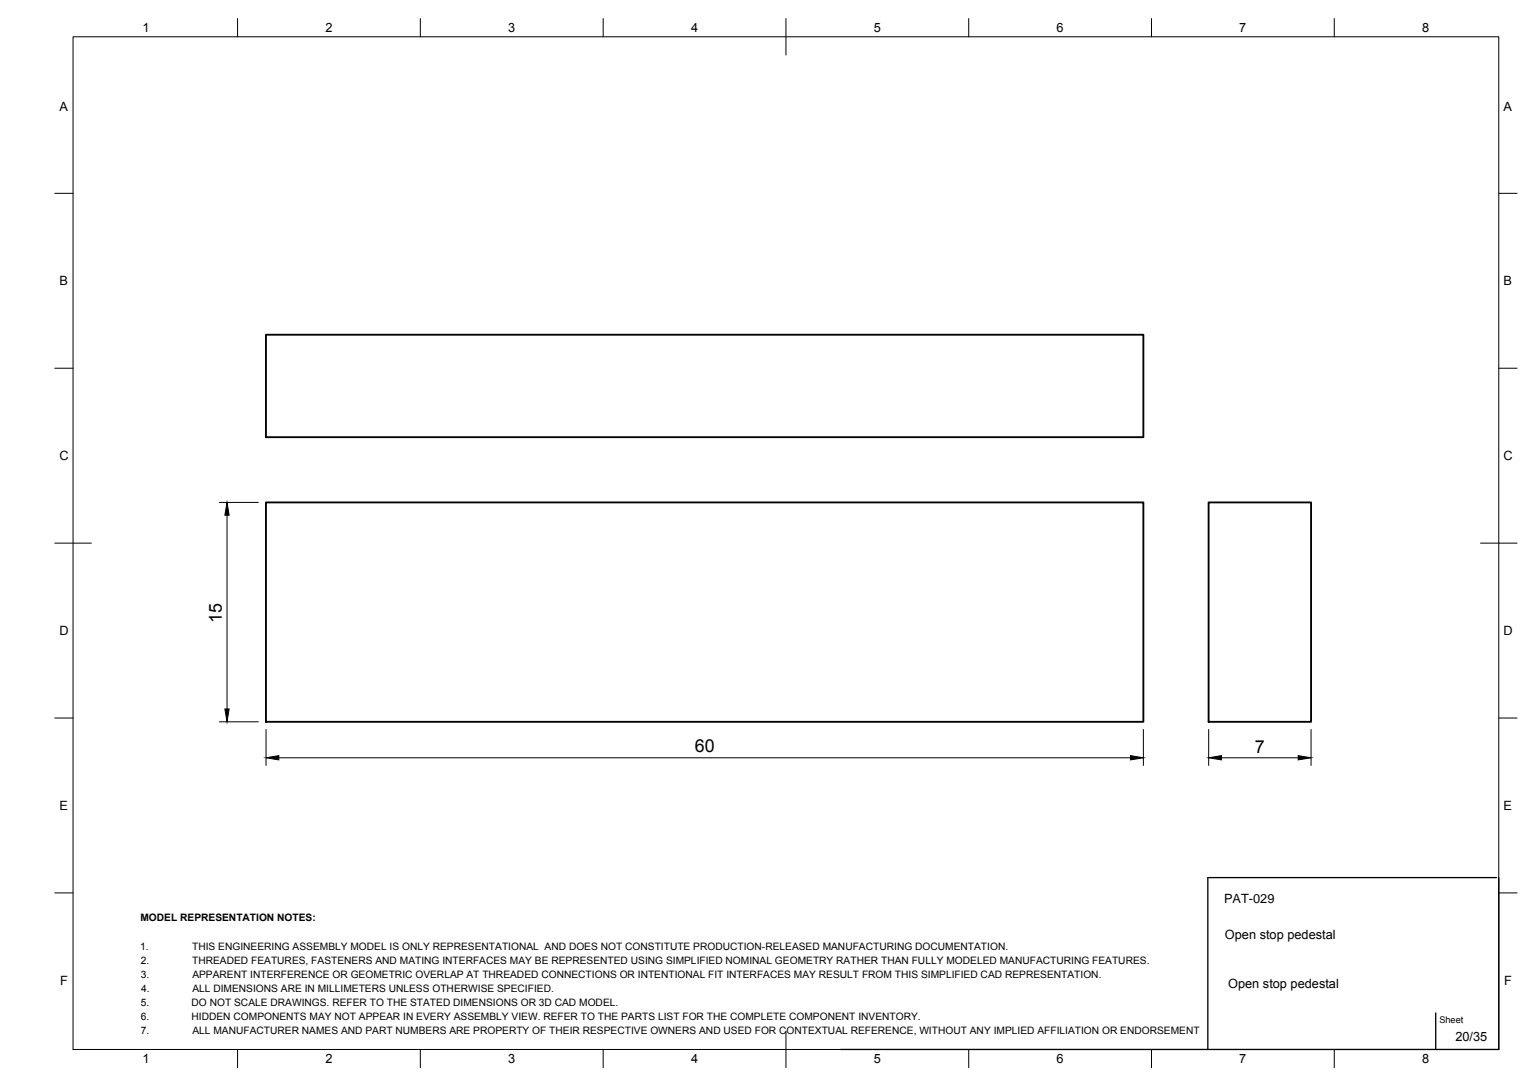
ISO-10303-21;
HEADER;
/* Generated by software containing ST-Developer
 * from STEP Tools, Inc. (www.steptools.com) 
 */

FILE_DESCRIPTION(
/* description */ ('Door-style hinge test fixture with detent'),
/* implementation_level */ '2;1');

FILE_NAME(
/* name */ 'Open stop pedestal.step',
/* time_stamp */ '2026-10-28T03:24:57-07:00',
/* author */ (''),
/* organization */ (''),
/* preprocessor_version */ 'ST-DEVELOPER v20.2',
/* originating_system */ 'Autodesk Translation Framework v15.17.0.0',
/* authorisation */ '');

FILE_SCHEMA (('AUTOMOTIVE_DESIGN { 1 0 10303 214 3 1 1 }'));
ENDSEC;

DATA;
#10=MECHANICAL_DESIGN_GEOMETRIC_PRESENTATION_REPRESENTATION('',(#338),#9813);
#275=SHAPE_REPRESENTATION_RELATIONSHIP('SRR','None',#9952,#306);
#306=ADVANCED_BREP_SHAPE_REPRESENTATION('',(#378),#9795);
#338=STYLED_ITEM('',(#10169),#378);
#378=MANIFOLD_SOLID_BREP('Body1',#4769);
#580=PLANE('',#5396);
#581=PLANE('',#5397);
#582=PLANE('',#5398);
#583=PLANE('',#5399);
#584=PLANE('',#5400);
#585=PLANE('',#5401);
#793=FACE_OUTER_BOUND('',#1144,.T.);
#794=FACE_OUTER_BOUND('',#1145,.T.);
#795=FACE_OUTER_BOUND('',#1146,.T.);
#796=FACE_OUTER_BOUND('',#1147,.T.);
#797=FACE_OUTER_BOUND('',#1148,.T.);
#798=FACE_OUTER_BOUND('',#1149,.T.);
#1144=EDGE_LOOP('',(#3779,#3780,#3781,#3782));
#1145=EDGE_LOOP('',(#3783,#3784,#3785,#3786));
#1146=EDGE_LOOP('',(#3787,#3788,#3789,#3790));
#1147=EDGE_LOOP('',(#3791,#3792,#3793,#3794));
#1148=EDGE_LOOP('',(#3795,#3796,#3797,#3798));
#1149=EDGE_LOOP('',(#3799,#3800,#3801,#3802));
#1508=LINE('',#8639,#1828);
#1509=LINE('',#8641,#1829);
#1510=LINE('',#8643,#1830);
#1511=LINE('',#8644,#1831);
#1512=LINE('',#8647,#1832);
#1513=LINE('',#8649,#1833);
#1514=LINE('',#8650,#1834);
#1515=LINE('',#8653,#1835);
#1516=LINE('',#8655,#1836);
#1517=LINE('',#8656,#1837);
#1518=LINE('',#8658,#1838);
#1519=LINE('',#8659,#1839);
#1828=VECTOR('',#6443,1.);
#1829=VECTOR('',#6444,1.);
#1830=VECTOR('',#6445,1.);
#1831=VECTOR('',#6446,1.);
#1832=VECTOR('',#6449,1.);
#1833=VECTOR('',#6450,1.);
#1834=VECTOR('',#6451,1.);
#1835=VECTOR('',#6454,1.);
#1836=VECTOR('',#6455,1.);
#1837=VECTOR('',#6456,1.);
#1838=VECTOR('',#6459,1.);
#1839=VECTOR('',#6460,1.);
#2413=VERTEX_POINT('',#8637);
#2414=VERTEX_POINT('',#8638);
#2415=VERTEX_POINT('',#8640);
#2416=VERTEX_POINT('',#8642);
#2417=VERTEX_POINT('',#8646);
#2418=VERTEX_POINT('',#8648);
#2419=VERTEX_POINT('',#8652);
#2420=VERTEX_POINT('',#8654);
#2906=EDGE_CURVE('',#2413,#2414,#1508,.T.);
#2907=EDGE_CURVE('',#2414,#2415,#1509,.T.);
#2908=EDGE_CURVE('',#2416,#2415,#1510,.T.);
#2909=EDGE_CURVE('',#2413,#2416,#1511,.T.);
#2910=EDGE_CURVE('',#2417,#2413,#1512,.T.);
#2911=EDGE_CURVE('',#2418,#2416,#1513,.T.);
#2912=EDGE_CURVE('',#2417,#2418,#1514,.T.);
#2913=EDGE_CURVE('',#2419,#2417,#1515,.T.);
#2914=EDGE_CURVE('',#2420,#2418,#1516,.T.);
#2915=EDGE_CURVE('',#2419,#2420,#1517,.T.);
#2916=EDGE_CURVE('',#2414,#2419,#1518,.T.);
#2917=EDGE_CURVE('',#2415,#2420,#1519,.T.);
#3779=ORIENTED_EDGE('',*,*,#2906,.T.);
#3780=ORIENTED_EDGE('',*,*,#2907,.T.);
#3781=ORIENTED_EDGE('',*,*,#2908,.F.);
#3782=ORIENTED_EDGE('',*,*,#2909,.F.);
#3783=ORIENTED_EDGE('',*,*,#2910,.T.);
#3784=ORIENTED_EDGE('',*,*,#2909,.T.);
#3785=ORIENTED_EDGE('',*,*,#2911,.F.);
#3786=ORIENTED_EDGE('',*,*,#2912,.F.);
#3787=ORIENTED_EDGE('',*,*,#2913,.T.);
#3788=ORIENTED_EDGE('',*,*,#2912,.T.);
#3789=ORIENTED_EDGE('',*,*,#2914,.F.);
#3790=ORIENTED_EDGE('',*,*,#2915,.F.);
#3791=ORIENTED_EDGE('',*,*,#2916,.T.);
#3792=ORIENTED_EDGE('',*,*,#2915,.T.);
#3793=ORIENTED_EDGE('',*,*,#2917,.F.);
#3794=ORIENTED_EDGE('',*,*,#2907,.F.);
#3795=ORIENTED_EDGE('',*,*,#2917,.T.);
#3796=ORIENTED_EDGE('',*,*,#2914,.T.);
#3797=ORIENTED_EDGE('',*,*,#2911,.T.);
#3798=ORIENTED_EDGE('',*,*,#2908,.T.);
#3799=ORIENTED_EDGE('',*,*,#2916,.F.);
#3800=ORIENTED_EDGE('',*,*,#2906,.F.);
#3801=ORIENTED_EDGE('',*,*,#2910,.F.);
#3802=ORIENTED_EDGE('',*,*,#2913,.F.);
#4598=ADVANCED_FACE('',(#793),#580,.T.);
#4599=ADVANCED_FACE('',(#794),#581,.T.);
#4600=ADVANCED_FACE('',(#795),#582,.T.);
#4601=ADVANCED_FACE('',(#796),#583,.T.);
#4602=ADVANCED_FACE('',(#797),#584,.T.);
#4603=ADVANCED_FACE('',(#798),#585,.F.);
#4769=CLOSED_SHELL('',(#4598,#4599,#4600,#4601,#4602,#4603));
#5395=AXIS2_PLACEMENT_3D('',#8635,#6439,#6440);
#5396=AXIS2_PLACEMENT_3D('',#8636,#6441,#6442);
#5397=AXIS2_PLACEMENT_3D('',#8645,#6447,#6448);
#5398=AXIS2_PLACEMENT_3D('',#8651,#6452,#6453);
#5399=AXIS2_PLACEMENT_3D('',#8657,#6457,#6458);
#5400=AXIS2_PLACEMENT_3D('',#8660,#6461,#6462);
#5401=AXIS2_PLACEMENT_3D('',#8661,#6463,#6464);
#6439=DIRECTION('axis',(0.,0.,1.));
#6440=DIRECTION('refdir',(1.,0.,0.));
#6441=DIRECTION('center_axis',(0.,1.,0.));
#6442=DIRECTION('ref_axis',(-1.,0.,0.));
#6443=DIRECTION('',(-1.,0.,0.));
#6444=DIRECTION('',(0.,0.,1.));
#6445=DIRECTION('',(-1.,0.,0.));
#6446=DIRECTION('',(0.,0.,1.));
#6447=DIRECTION('center_axis',(1.,0.,0.));
#6448=DIRECTION('ref_axis',(0.,1.,0.));
#6449=DIRECTION('',(0.,1.,0.));
#6450=DIRECTION('',(0.,1.,0.));
#6451=DIRECTION('',(0.,0.,1.));
#6452=DIRECTION('center_axis',(0.,-1.,0.));
#6453=DIRECTION('ref_axis',(1.,0.,0.));
#6454=DIRECTION('',(1.,0.,0.));
#6455=DIRECTION('',(1.,0.,0.));
#6456=DIRECTION('',(0.,0.,1.));
#6457=DIRECTION('center_axis',(-1.,0.,0.));
#6458=DIRECTION('ref_axis',(0.,-1.,0.));
#6459=DIRECTION('',(0.,-1.,0.));
#6460=DIRECTION('',(0.,-1.,0.));
#6461=DIRECTION('center_axis',(0.,0.,1.));
#6462=DIRECTION('ref_axis',(1.,0.,0.));
#6463=DIRECTION('center_axis',(0.,0.,1.));
#6464=DIRECTION('ref_axis',(1.,0.,0.));
#8635=CARTESIAN_POINT('',(0.,0.,0.));
#8636=CARTESIAN_POINT('Origin',(-0.6,11.,0.));
#8637=CARTESIAN_POINT('',(-0.6,11.,0.));
#8638=CARTESIAN_POINT('',(-1.3,11.,0.));
#8639=CARTESIAN_POINT('',(-0.6,11.,0.));
#8640=CARTESIAN_POINT('',(-1.3,11.,6.));
#8641=CARTESIAN_POINT('',(-1.3,11.,0.));
#8642=CARTESIAN_POINT('',(-0.6,11.,6.));
#8643=CARTESIAN_POINT('',(-0.6,11.,6.));
#8644=CARTESIAN_POINT('',(-0.6,11.,0.));
#8645=CARTESIAN_POINT('Origin',(-0.6,9.5,0.));
#8646=CARTESIAN_POINT('',(-0.6,9.5,0.));
#8647=CARTESIAN_POINT('',(-0.6,9.5,0.));
#8648=CARTESIAN_POINT('',(-0.6,9.5,6.));
#8649=CARTESIAN_POINT('',(-0.6,9.5,6.));
#8650=CARTESIAN_POINT('',(-0.6,9.5,0.));
#8651=CARTESIAN_POINT('Origin',(-1.3,9.5,0.));
#8652=CARTESIAN_POINT('',(-1.3,9.5,0.));
#8653=CARTESIAN_POINT('',(-1.3,9.5,0.));
#8654=CARTESIAN_POINT('',(-1.3,9.5,6.));
#8655=CARTESIAN_POINT('',(-1.3,9.5,6.));
#8656=CARTESIAN_POINT('',(-1.3,9.5,0.));
#8657=CARTESIAN_POINT('Origin',(-1.3,11.,0.));
#8658=CARTESIAN_POINT('',(-1.3,11.,0.));
#8659=CARTESIAN_POINT('',(-1.3,11.,6.));
#8660=CARTESIAN_POINT('Origin',(-0.95,10.25,6.));
#8661=CARTESIAN_POINT('Origin',(-0.95,10.25,0.));
#9759=UNCERTAINTY_MEASURE_WITH_UNIT(LENGTH_MEASURE(0.001),#9814,
'DISTANCE_ACCURACY_VALUE',
'Maximum model space distance between geometric entities at asserted c
onnectivities');
#9777=UNCERTAINTY_MEASURE_WITH_UNIT(LENGTH_MEASURE(0.001),#9814,
'DISTANCE_ACCURACY_VALUE',
'Maximum model space distance between geometric entities at asserted c
onnectivities');
#9795=(
GEOMETRIC_REPRESENTATION_CONTEXT(3)
GLOBAL_UNCERTAINTY_ASSIGNED_CONTEXT((#9759))
GLOBAL_UNIT_ASSIGNED_CONTEXT((#9814,#9816,#9817))
REPRESENTATION_CONTEXT('','3D')
);
#9813=(
GEOMETRIC_REPRESENTATION_CONTEXT(3)
GLOBAL_UNCERTAINTY_ASSIGNED_CONTEXT((#9777))
GLOBAL_UNIT_ASSIGNED_CONTEXT((#9814,#9816,#9817))
REPRESENTATION_CONTEXT('','3D')
);
#9814=(
LENGTH_UNIT()
NAMED_UNIT(*)
SI_UNIT(.CENTI.,.METRE.)
);
#9816=(
NAMED_UNIT(*)
PLANE_ANGLE_UNIT()
SI_UNIT($,.RADIAN.)
);
#9817=(
NAMED_UNIT(*)
SI_UNIT($,.STERADIAN.)
SOLID_ANGLE_UNIT()
);
#9835=SHAPE_DEFINITION_REPRESENTATION(#9870,#9952);
#9870=PRODUCT_DEFINITION_SHAPE('',$,#9988);
#9952=SHAPE_REPRESENTATION('',(#5395),#9795);
#9970=PRODUCT_DEFINITION_CONTEXT('part definition',#10077,'design');
#9988=PRODUCT_DEFINITION('Open stop pedestal','Open stop pedestal',#10023,
#9970);
#10023=PRODUCT_DEFINITION_FORMATION('',$,#10096);
#10077=APPLICATION_CONTEXT(
'Core Data for Automotive Mechanical Design Process');
#10078=PRODUCT_CONTEXT('part definition',#10077,'mechanical');
#10096=PRODUCT('Open stop pedestal','Open stop pedestal',
'Open stop pedestal',(#10078));
#10163=COLOUR_RGB('Light Blue',0.38,0.62,0.78);
#10164=FILL_AREA_STYLE_COLOUR('',#10163);
#10165=FILL_AREA_STYLE('',(#10164));
#10166=SURFACE_STYLE_FILL_AREA(#10165);
#10167=SURFACE_SIDE_STYLE('',(#10166));
#10168=SURFACE_STYLE_USAGE(.BOTH.,#10167);
#10169=PRESENTATION_STYLE_ASSIGNMENT((#10168));
ENDSEC;
END-ISO-10303-21;
